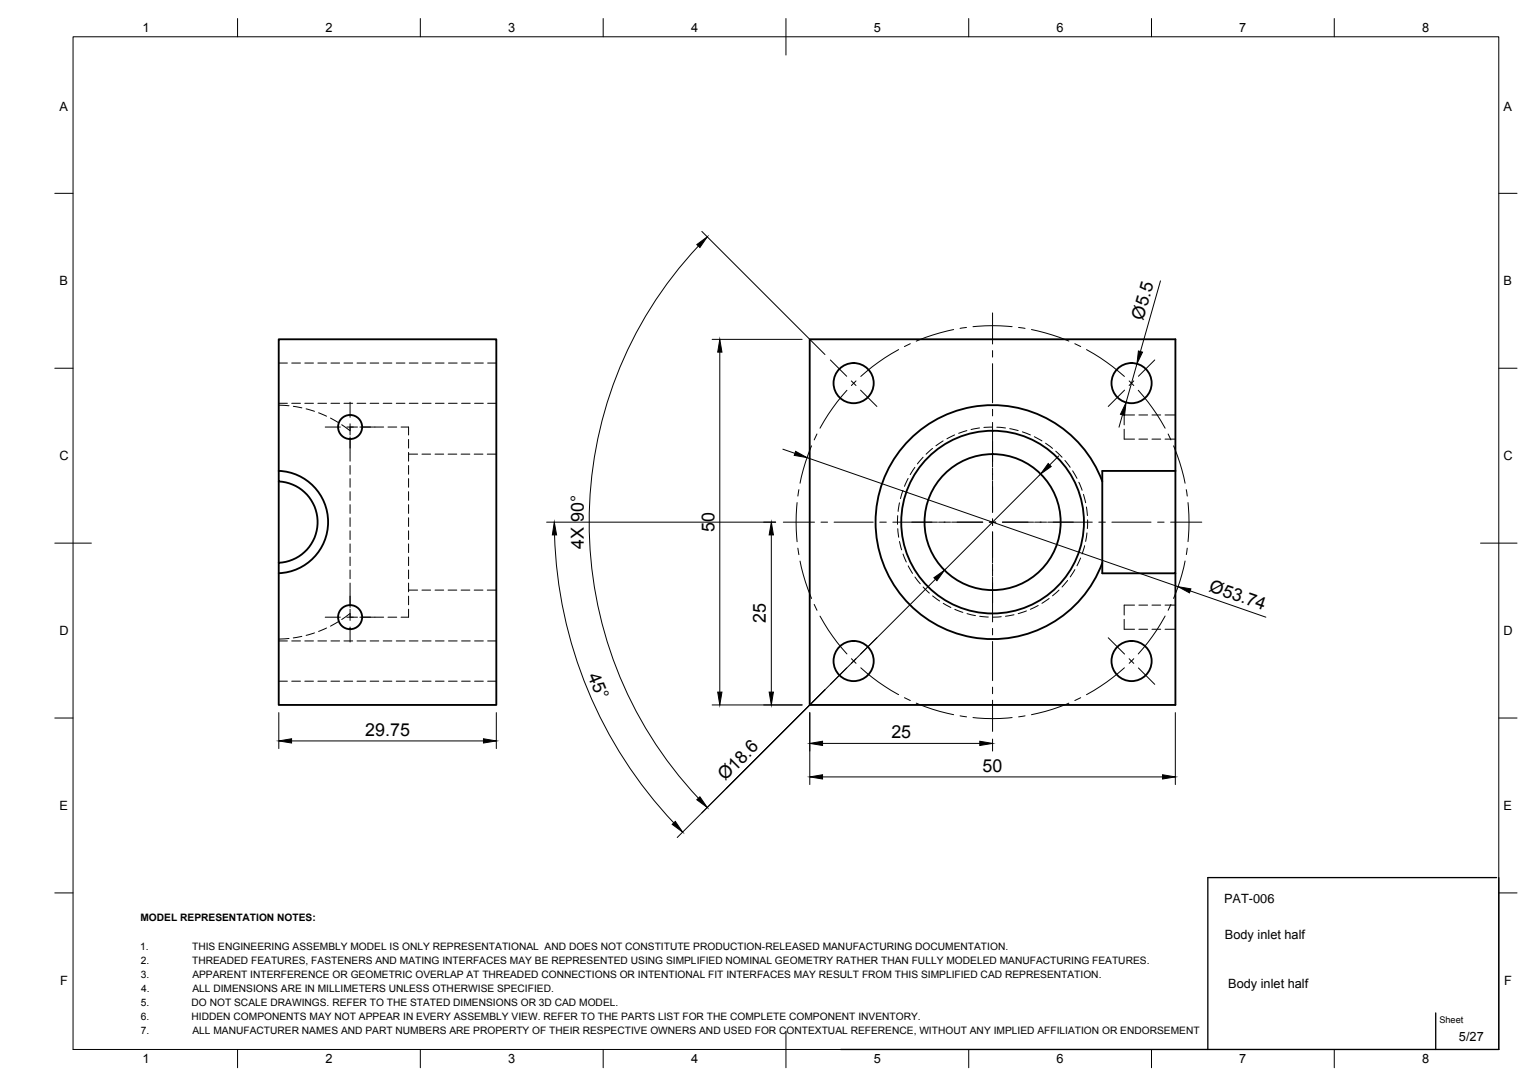
ISO-10303-21;
HEADER;
/* Generated by software containing ST-Developer
 * from STEP Tools, Inc. (www.steptools.com) 
 */

FILE_DESCRIPTION(
/* description */ ('Ball-type isolation valve (generic)'),
/* implementation_level */ '2;1');

FILE_NAME(
/* name */ 'Body inlet half.step',
/* time_stamp */ '2026-10-27T10:53:05-07:00',
/* author */ (''),
/* organization */ (''),
/* preprocessor_version */ 'ST-DEVELOPER v20.2',
/* originating_system */ 'Autodesk Translation Framework v15.17.0.0',
/* authorisation */ '');

FILE_SCHEMA (('AUTOMOTIVE_DESIGN { 1 0 10303 214 3 1 1 }'));
ENDSEC;

DATA;
#10=MECHANICAL_DESIGN_GEOMETRIC_PRESENTATION_REPRESENTATION('',(#277),#7425);
#225=SHAPE_REPRESENTATION_RELATIONSHIP('SRR','None',#7535,#251);
#251=ADVANCED_BREP_SHAPE_REPRESENTATION('',(#303),#7398);
#277=STYLED_ITEM('',(#7723),#303);
#303=MANIFOLD_SOLID_BREP('Body1',#4082);
#326=SPHERICAL_SURFACE('',#4436,1.6);
#331=FACE_BOUND('',#839,.T.);
#332=FACE_BOUND('',#840,.T.);
#333=FACE_BOUND('',#844,.T.);
#334=FACE_BOUND('',#846,.T.);
#335=FACE_BOUND('',#848,.T.);
#336=FACE_BOUND('',#850,.T.);
#337=FACE_BOUND('',#851,.T.);
#338=FACE_BOUND('',#852,.T.);
#339=FACE_BOUND('',#853,.T.);
#340=FACE_BOUND('',#856,.T.);
#341=FACE_BOUND('',#857,.T.);
#342=FACE_BOUND('',#858,.T.);
#343=FACE_BOUND('',#859,.T.);
#344=FACE_BOUND('',#860,.T.);
#419=PLANE('',#4404);
#420=PLANE('',#4408);
#421=PLANE('',#4424);
#422=PLANE('',#4426);
#423=PLANE('',#4433);
#424=PLANE('',#4435);
#425=PLANE('',#4438);
#426=PLANE('',#4439);
#427=PLANE('',#4440);
#428=PLANE('',#4441);
#429=PLANE('',#4442);
#579=FACE_OUTER_BOUND('',#828,.T.);
#580=FACE_OUTER_BOUND('',#829,.T.);
#581=FACE_OUTER_BOUND('',#830,.T.);
#582=FACE_OUTER_BOUND('',#831,.T.);
#583=FACE_OUTER_BOUND('',#832,.T.);
#584=FACE_OUTER_BOUND('',#833,.T.);
#585=FACE_OUTER_BOUND('',#834,.T.);
#586=FACE_OUTER_BOUND('',#835,.T.);
#587=FACE_OUTER_BOUND('',#836,.T.);
#588=FACE_OUTER_BOUND('',#837,.T.);
#589=FACE_OUTER_BOUND('',#838,.T.);
#590=FACE_OUTER_BOUND('',#841,.T.);
#591=FACE_OUTER_BOUND('',#842,.T.);
#592=FACE_OUTER_BOUND('',#843,.T.);
#593=FACE_OUTER_BOUND('',#845,.T.);
#594=FACE_OUTER_BOUND('',#847,.T.);
#595=FACE_OUTER_BOUND('',#849,.T.);
#596=FACE_OUTER_BOUND('',#854,.T.);
#597=FACE_OUTER_BOUND('',#855,.T.);
#598=FACE_OUTER_BOUND('',#861,.T.);
#599=FACE_OUTER_BOUND('',#862,.T.);
#828=EDGE_LOOP('',(#2775,#2776,#2777,#2778));
#829=EDGE_LOOP('',(#2779));
#830=EDGE_LOOP('',(#2780,#2781,#2782,#2783));
#831=EDGE_LOOP('',(#2784));
#832=EDGE_LOOP('',(#2785,#2786,#2787,#2788));
#833=EDGE_LOOP('',(#2789,#2790,#2791,#2792));
#834=EDGE_LOOP('',(#2793,#2794,#2795,#2796));
#835=EDGE_LOOP('',(#2797,#2798,#2799,#2800));
#836=EDGE_LOOP('',(#2801,#2802,#2803,#2804));
#837=EDGE_LOOP('',(#2805,#2806,#2807,#2808));
#838=EDGE_LOOP('',(#2809,#2810,#2811,#2812,#2813,#2814));
#839=EDGE_LOOP('',(#2815));
#840=EDGE_LOOP('',(#2816));
#841=EDGE_LOOP('',(#2817,#2818,#2819,#2820));
#842=EDGE_LOOP('',(#2821,#2822,#2823,#2824));
#843=EDGE_LOOP('',(#2825));
#844=EDGE_LOOP('',(#2826));
#845=EDGE_LOOP('',(#2827));
#846=EDGE_LOOP('',(#2828));
#847=EDGE_LOOP('',(#2829,#2830));
#848=EDGE_LOOP('',(#2831));
#849=EDGE_LOOP('',(#2832,#2833,#2834,#2835,#2836,#2837,#2838,#2839,#2840,
#2841));
#850=EDGE_LOOP('',(#2842));
#851=EDGE_LOOP('',(#2843));
#852=EDGE_LOOP('',(#2844));
#853=EDGE_LOOP('',(#2845));
#854=EDGE_LOOP('',(#2846,#2847,#2848,#2849));
#855=EDGE_LOOP('',(#2850,#2851,#2852,#2853));
#856=EDGE_LOOP('',(#2854));
#857=EDGE_LOOP('',(#2855));
#858=EDGE_LOOP('',(#2856));
#859=EDGE_LOOP('',(#2857));
#860=EDGE_LOOP('',(#2858));
#861=EDGE_LOOP('',(#2859,#2860,#2861,#2862));
#862=EDGE_LOOP('',(#2863,#2864,#2865,#2866));
#1165=LINE('',#6207,#1473);
#1166=LINE('',#6214,#1474);
#1167=LINE('',#6221,#1475);
#1168=LINE('',#6227,#1476);
#1169=LINE('',#6233,#1477);
#1170=LINE('',#6239,#1478);
#1171=LINE('',#6244,#1479);
#1172=LINE('',#6248,#1480);
#1173=LINE('',#6252,#1481);
#1174=LINE('',#6255,#1482);
#1175=LINE('',#6258,#1483);
#1176=LINE('',#6260,#1484);
#1177=LINE('',#6262,#1485);
#1178=LINE('',#6264,#1486);
#1179=LINE('',#6265,#1487);
#1180=LINE('',#6270,#1488);
#1181=LINE('',#6276,#1489);
#1182=LINE('',#6286,#1490);
#1183=LINE('',#6288,#1491);
#1184=LINE('',#6289,#1492);
#1185=LINE('',#6292,#1493);
#1186=LINE('',#6293,#1494);
#1187=LINE('',#6296,#1495);
#1188=LINE('',#6297,#1496);
#1189=LINE('',#6299,#1497);
#1473=VECTOR('',#4906,0.165);
#1474=VECTOR('',#4915,0.165);
#1475=VECTOR('',#4924,0.275);
#1476=VECTOR('',#4931,0.275);
#1477=VECTOR('',#4938,0.275);
#1478=VECTOR('',#4945,0.275);
#1479=VECTOR('',#4950,1.);
#1480=VECTOR('',#4953,1.);
#1481=VECTOR('',#4958,1.);
#1482=VECTOR('',#4961,1.);
#1483=VECTOR('',#4964,1.);
#1484=VECTOR('',#4965,1.);
#1485=VECTOR('',#4966,1.);
#1486=VECTOR('',#4967,1.);
#1487=VECTOR('',#4968,1.);
#1488=VECTOR('',#4973,0.93);
#1489=VECTOR('',#4980,1.3);
#1490=VECTOR('',#4995,1.);
#1491=VECTOR('',#4996,1.);
#1492=VECTOR('',#4997,1.);
#1493=VECTOR('',#5000,1.);
#1494=VECTOR('',#5001,1.);
#1495=VECTOR('',#5004,1.);
#1496=VECTOR('',#5005,1.);
#1497=VECTOR('',#5008,1.);
#1781=CIRCLE('',#4402,0.165);
#1782=CIRCLE('',#4403,0.165);
#1783=CIRCLE('',#4406,0.165);
#1784=CIRCLE('',#4407,0.165);
#1785=CIRCLE('',#4410,0.275);
#1786=CIRCLE('',#4411,0.275);
#1787=CIRCLE('',#4413,0.275);
#1788=CIRCLE('',#4414,0.275);
#1789=CIRCLE('',#4416,0.275);
#1790=CIRCLE('',#4417,0.275);
#1791=CIRCLE('',#4419,0.275);
#1792=CIRCLE('',#4420,0.275);
#1793=CIRCLE('',#4422,0.7);
#1794=CIRCLE('',#4423,0.7);
#1795=CIRCLE('',#4425,0.556776436283003);
#1796=CIRCLE('',#4428,0.93);
#1797=CIRCLE('',#4429,0.93);
#1798=CIRCLE('',#4431,1.3);
#1799=CIRCLE('',#4432,1.3);
#1800=CIRCLE('',#4434,1.24899959967968);
#1801=CIRCLE('',#4437,1.59980467557762);
#1956=VERTEX_POINT('',#6204);
#1957=VERTEX_POINT('',#6206);
#1958=VERTEX_POINT('',#6211);
#1959=VERTEX_POINT('',#6213);
#1960=VERTEX_POINT('',#6218);
#1961=VERTEX_POINT('',#6220);
#1962=VERTEX_POINT('',#6224);
#1963=VERTEX_POINT('',#6226);
#1964=VERTEX_POINT('',#6230);
#1965=VERTEX_POINT('',#6232);
#1966=VERTEX_POINT('',#6236);
#1967=VERTEX_POINT('',#6238);
#1968=VERTEX_POINT('',#6242);
#1969=VERTEX_POINT('',#6243);
#1970=VERTEX_POINT('',#6245);
#1971=VERTEX_POINT('',#6247);
#1972=VERTEX_POINT('',#6251);
#1973=VERTEX_POINT('',#6253);
#1974=VERTEX_POINT('',#6257);
#1975=VERTEX_POINT('',#6259);
#1976=VERTEX_POINT('',#6261);
#1977=VERTEX_POINT('',#6263);
#1978=VERTEX_POINT('',#6267);
#1979=VERTEX_POINT('',#6269);
#1980=VERTEX_POINT('',#6273);
#1981=VERTEX_POINT('',#6275);
#1982=VERTEX_POINT('',#6279);
#1983=VERTEX_POINT('',#6285);
#1984=VERTEX_POINT('',#6287);
#1985=VERTEX_POINT('',#6291);
#1986=VERTEX_POINT('',#6295);
#2280=EDGE_CURVE('',#1956,#1956,#1781,.T.);
#2281=EDGE_CURVE('',#1956,#1957,#1165,.T.);
#2282=EDGE_CURVE('',#1957,#1957,#1782,.T.);
#2283=EDGE_CURVE('',#1958,#1958,#1783,.T.);
#2284=EDGE_CURVE('',#1958,#1959,#1166,.T.);
#2285=EDGE_CURVE('',#1959,#1959,#1784,.T.);
#2286=EDGE_CURVE('',#1960,#1960,#1785,.T.);
#2287=EDGE_CURVE('',#1960,#1961,#1167,.T.);
#2288=EDGE_CURVE('',#1961,#1961,#1786,.T.);
#2289=EDGE_CURVE('',#1962,#1962,#1787,.T.);
#2290=EDGE_CURVE('',#1962,#1963,#1168,.T.);
#2291=EDGE_CURVE('',#1963,#1963,#1788,.T.);
#2292=EDGE_CURVE('',#1964,#1964,#1789,.T.);
#2293=EDGE_CURVE('',#1964,#1965,#1169,.T.);
#2294=EDGE_CURVE('',#1965,#1965,#1790,.T.);
#2295=EDGE_CURVE('',#1966,#1966,#1791,.T.);
#2296=EDGE_CURVE('',#1966,#1967,#1170,.T.);
#2297=EDGE_CURVE('',#1967,#1967,#1792,.T.);
#2298=EDGE_CURVE('',#1968,#1969,#1171,.T.);
#2299=EDGE_CURVE('',#1970,#1968,#1793,.T.);
#2300=EDGE_CURVE('',#1971,#1970,#1172,.T.);
#2301=EDGE_CURVE('',#1969,#1971,#1794,.T.);
#2302=EDGE_CURVE('',#1972,#1968,#1173,.T.);
#2303=EDGE_CURVE('',#1973,#1972,#1795,.T.);
#2304=EDGE_CURVE('',#1970,#1973,#1174,.T.);
#2305=EDGE_CURVE('',#1971,#1974,#1175,.T.);
#2306=EDGE_CURVE('',#1974,#1975,#1176,.T.);
#2307=EDGE_CURVE('',#1975,#1976,#1177,.T.);
#2308=EDGE_CURVE('',#1976,#1977,#1178,.T.);
#2309=EDGE_CURVE('',#1977,#1969,#1179,.T.);
#2310=EDGE_CURVE('',#1978,#1978,#1796,.T.);
#2311=EDGE_CURVE('',#1978,#1979,#1180,.T.);
#2312=EDGE_CURVE('',#1979,#1979,#1797,.T.);
#2313=EDGE_CURVE('',#1980,#1980,#1798,.T.);
#2314=EDGE_CURVE('',#1980,#1981,#1181,.T.);
#2315=EDGE_CURVE('',#1981,#1981,#1799,.T.);
#2316=EDGE_CURVE('',#1982,#1982,#1800,.T.);
#2317=EDGE_CURVE('',#1973,#1972,#1801,.T.);
#2318=EDGE_CURVE('',#1983,#1977,#1182,.T.);
#2319=EDGE_CURVE('',#1983,#1984,#1183,.T.);
#2320=EDGE_CURVE('',#1984,#1974,#1184,.T.);
#2321=EDGE_CURVE('',#1985,#1983,#1185,.T.);
#2322=EDGE_CURVE('',#1985,#1976,#1186,.T.);
#2323=EDGE_CURVE('',#1986,#1985,#1187,.T.);
#2324=EDGE_CURVE('',#1986,#1975,#1188,.T.);
#2325=EDGE_CURVE('',#1984,#1986,#1189,.T.);
#2775=ORIENTED_EDGE('',*,*,#2280,.F.);
#2776=ORIENTED_EDGE('',*,*,#2281,.T.);
#2777=ORIENTED_EDGE('',*,*,#2282,.F.);
#2778=ORIENTED_EDGE('',*,*,#2281,.F.);
#2779=ORIENTED_EDGE('',*,*,#2280,.T.);
#2780=ORIENTED_EDGE('',*,*,#2283,.F.);
#2781=ORIENTED_EDGE('',*,*,#2284,.T.);
#2782=ORIENTED_EDGE('',*,*,#2285,.F.);
#2783=ORIENTED_EDGE('',*,*,#2284,.F.);
#2784=ORIENTED_EDGE('',*,*,#2283,.T.);
#2785=ORIENTED_EDGE('',*,*,#2286,.F.);
#2786=ORIENTED_EDGE('',*,*,#2287,.T.);
#2787=ORIENTED_EDGE('',*,*,#2288,.F.);
#2788=ORIENTED_EDGE('',*,*,#2287,.F.);
#2789=ORIENTED_EDGE('',*,*,#2289,.F.);
#2790=ORIENTED_EDGE('',*,*,#2290,.T.);
#2791=ORIENTED_EDGE('',*,*,#2291,.F.);
#2792=ORIENTED_EDGE('',*,*,#2290,.F.);
#2793=ORIENTED_EDGE('',*,*,#2292,.F.);
#2794=ORIENTED_EDGE('',*,*,#2293,.T.);
#2795=ORIENTED_EDGE('',*,*,#2294,.F.);
#2796=ORIENTED_EDGE('',*,*,#2293,.F.);
#2797=ORIENTED_EDGE('',*,*,#2295,.F.);
#2798=ORIENTED_EDGE('',*,*,#2296,.T.);
#2799=ORIENTED_EDGE('',*,*,#2297,.F.);
#2800=ORIENTED_EDGE('',*,*,#2296,.F.);
#2801=ORIENTED_EDGE('',*,*,#2298,.F.);
#2802=ORIENTED_EDGE('',*,*,#2299,.F.);
#2803=ORIENTED_EDGE('',*,*,#2300,.F.);
#2804=ORIENTED_EDGE('',*,*,#2301,.F.);
#2805=ORIENTED_EDGE('',*,*,#2302,.F.);
#2806=ORIENTED_EDGE('',*,*,#2303,.F.);
#2807=ORIENTED_EDGE('',*,*,#2304,.F.);
#2808=ORIENTED_EDGE('',*,*,#2299,.T.);
#2809=ORIENTED_EDGE('',*,*,#2301,.T.);
#2810=ORIENTED_EDGE('',*,*,#2305,.T.);
#2811=ORIENTED_EDGE('',*,*,#2306,.T.);
#2812=ORIENTED_EDGE('',*,*,#2307,.T.);
#2813=ORIENTED_EDGE('',*,*,#2308,.T.);
#2814=ORIENTED_EDGE('',*,*,#2309,.T.);
#2815=ORIENTED_EDGE('',*,*,#2282,.T.);
#2816=ORIENTED_EDGE('',*,*,#2285,.T.);
#2817=ORIENTED_EDGE('',*,*,#2310,.F.);
#2818=ORIENTED_EDGE('',*,*,#2311,.T.);
#2819=ORIENTED_EDGE('',*,*,#2312,.F.);
#2820=ORIENTED_EDGE('',*,*,#2311,.F.);
#2821=ORIENTED_EDGE('',*,*,#2313,.F.);
#2822=ORIENTED_EDGE('',*,*,#2314,.T.);
#2823=ORIENTED_EDGE('',*,*,#2315,.T.);
#2824=ORIENTED_EDGE('',*,*,#2314,.F.);
#2825=ORIENTED_EDGE('',*,*,#2315,.F.);
#2826=ORIENTED_EDGE('',*,*,#2316,.F.);
#2827=ORIENTED_EDGE('',*,*,#2313,.T.);
#2828=ORIENTED_EDGE('',*,*,#2312,.T.);
#2829=ORIENTED_EDGE('',*,*,#2303,.T.);
#2830=ORIENTED_EDGE('',*,*,#2317,.F.);
#2831=ORIENTED_EDGE('',*,*,#2316,.T.);
#2832=ORIENTED_EDGE('',*,*,#2298,.T.);
#2833=ORIENTED_EDGE('',*,*,#2309,.F.);
#2834=ORIENTED_EDGE('',*,*,#2318,.F.);
#2835=ORIENTED_EDGE('',*,*,#2319,.T.);
#2836=ORIENTED_EDGE('',*,*,#2320,.T.);
#2837=ORIENTED_EDGE('',*,*,#2305,.F.);
#2838=ORIENTED_EDGE('',*,*,#2300,.T.);
#2839=ORIENTED_EDGE('',*,*,#2304,.T.);
#2840=ORIENTED_EDGE('',*,*,#2317,.T.);
#2841=ORIENTED_EDGE('',*,*,#2302,.T.);
#2842=ORIENTED_EDGE('',*,*,#2288,.T.);
#2843=ORIENTED_EDGE('',*,*,#2291,.T.);
#2844=ORIENTED_EDGE('',*,*,#2294,.T.);
#2845=ORIENTED_EDGE('',*,*,#2297,.T.);
#2846=ORIENTED_EDGE('',*,*,#2321,.T.);
#2847=ORIENTED_EDGE('',*,*,#2318,.T.);
#2848=ORIENTED_EDGE('',*,*,#2308,.F.);
#2849=ORIENTED_EDGE('',*,*,#2322,.F.);
#2850=ORIENTED_EDGE('',*,*,#2323,.T.);
#2851=ORIENTED_EDGE('',*,*,#2322,.T.);
#2852=ORIENTED_EDGE('',*,*,#2307,.F.);
#2853=ORIENTED_EDGE('',*,*,#2324,.F.);
#2854=ORIENTED_EDGE('',*,*,#2310,.T.);
#2855=ORIENTED_EDGE('',*,*,#2295,.T.);
#2856=ORIENTED_EDGE('',*,*,#2292,.T.);
#2857=ORIENTED_EDGE('',*,*,#2289,.T.);
#2858=ORIENTED_EDGE('',*,*,#2286,.T.);
#2859=ORIENTED_EDGE('',*,*,#2325,.T.);
#2860=ORIENTED_EDGE('',*,*,#2324,.T.);
#2861=ORIENTED_EDGE('',*,*,#2306,.F.);
#2862=ORIENTED_EDGE('',*,*,#2320,.F.);
#2863=ORIENTED_EDGE('',*,*,#2325,.F.);
#2864=ORIENTED_EDGE('',*,*,#2319,.F.);
#2865=ORIENTED_EDGE('',*,*,#2321,.F.);
#2866=ORIENTED_EDGE('',*,*,#2323,.F.);
#3765=CYLINDRICAL_SURFACE('',#4401,0.165);
#3766=CYLINDRICAL_SURFACE('',#4405,0.165);
#3767=CYLINDRICAL_SURFACE('',#4409,0.275);
#3768=CYLINDRICAL_SURFACE('',#4412,0.275);
#3769=CYLINDRICAL_SURFACE('',#4415,0.275);
#3770=CYLINDRICAL_SURFACE('',#4418,0.275);
#3771=CYLINDRICAL_SURFACE('',#4421,0.7);
#3772=CYLINDRICAL_SURFACE('',#4427,0.93);
#3773=CYLINDRICAL_SURFACE('',#4430,1.3);
#3833=ADVANCED_FACE('',(#579),#3765,.F.);
#3834=ADVANCED_FACE('',(#580),#419,.T.);
#3835=ADVANCED_FACE('',(#581),#3766,.F.);
#3836=ADVANCED_FACE('',(#582),#420,.T.);
#3837=ADVANCED_FACE('',(#583),#3767,.F.);
#3838=ADVANCED_FACE('',(#584),#3768,.F.);
#3839=ADVANCED_FACE('',(#585),#3769,.F.);
#3840=ADVANCED_FACE('',(#586),#3770,.F.);
#3841=ADVANCED_FACE('',(#587),#3771,.F.);
#3842=ADVANCED_FACE('',(#588),#421,.T.);
#3843=ADVANCED_FACE('',(#589,#331,#332),#422,.T.);
#3844=ADVANCED_FACE('',(#590),#3772,.F.);
#3845=ADVANCED_FACE('',(#591),#3773,.F.);
#3846=ADVANCED_FACE('',(#592,#333),#423,.F.);
#3847=ADVANCED_FACE('',(#593,#334),#424,.T.);
#3848=ADVANCED_FACE('',(#594,#335),#326,.F.);
#3849=ADVANCED_FACE('',(#595,#336,#337,#338,#339),#425,.T.);
#3850=ADVANCED_FACE('',(#596),#426,.T.);
#3851=ADVANCED_FACE('',(#597,#340,#341,#342,#343,#344),#427,.T.);
#3852=ADVANCED_FACE('',(#598),#428,.T.);
#3853=ADVANCED_FACE('',(#599),#429,.F.);
#4082=CLOSED_SHELL('',(#3833,#3834,#3835,#3836,#3837,#3838,#3839,#3840,
#3841,#3842,#3843,#3844,#3845,#3846,#3847,#3848,#3849,#3850,#3851,#3852,
#3853));
#4400=AXIS2_PLACEMENT_3D('',#6202,#4900,#4901);
#4401=AXIS2_PLACEMENT_3D('',#6203,#4902,#4903);
#4402=AXIS2_PLACEMENT_3D('',#6205,#4904,#4905);
#4403=AXIS2_PLACEMENT_3D('',#6208,#4907,#4908);
#4404=AXIS2_PLACEMENT_3D('',#6209,#4909,#4910);
#4405=AXIS2_PLACEMENT_3D('',#6210,#4911,#4912);
#4406=AXIS2_PLACEMENT_3D('',#6212,#4913,#4914);
#4407=AXIS2_PLACEMENT_3D('',#6215,#4916,#4917);
#4408=AXIS2_PLACEMENT_3D('',#6216,#4918,#4919);
#4409=AXIS2_PLACEMENT_3D('',#6217,#4920,#4921);
#4410=AXIS2_PLACEMENT_3D('',#6219,#4922,#4923);
#4411=AXIS2_PLACEMENT_3D('',#6222,#4925,#4926);
#4412=AXIS2_PLACEMENT_3D('',#6223,#4927,#4928);
#4413=AXIS2_PLACEMENT_3D('',#6225,#4929,#4930);
#4414=AXIS2_PLACEMENT_3D('',#6228,#4932,#4933);
#4415=AXIS2_PLACEMENT_3D('',#6229,#4934,#4935);
#4416=AXIS2_PLACEMENT_3D('',#6231,#4936,#4937);
#4417=AXIS2_PLACEMENT_3D('',#6234,#4939,#4940);
#4418=AXIS2_PLACEMENT_3D('',#6235,#4941,#4942);
#4419=AXIS2_PLACEMENT_3D('',#6237,#4943,#4944);
#4420=AXIS2_PLACEMENT_3D('',#6240,#4946,#4947);
#4421=AXIS2_PLACEMENT_3D('',#6241,#4948,#4949);
#4422=AXIS2_PLACEMENT_3D('',#6246,#4951,#4952);
#4423=AXIS2_PLACEMENT_3D('',#6249,#4954,#4955);
#4424=AXIS2_PLACEMENT_3D('',#6250,#4956,#4957);
#4425=AXIS2_PLACEMENT_3D('',#6254,#4959,#4960);
#4426=AXIS2_PLACEMENT_3D('',#6256,#4962,#4963);
#4427=AXIS2_PLACEMENT_3D('',#6266,#4969,#4970);
#4428=AXIS2_PLACEMENT_3D('',#6268,#4971,#4972);
#4429=AXIS2_PLACEMENT_3D('',#6271,#4974,#4975);
#4430=AXIS2_PLACEMENT_3D('',#6272,#4976,#4977);
#4431=AXIS2_PLACEMENT_3D('',#6274,#4978,#4979);
#4432=AXIS2_PLACEMENT_3D('',#6277,#4981,#4982);
#4433=AXIS2_PLACEMENT_3D('',#6278,#4983,#4984);
#4434=AXIS2_PLACEMENT_3D('',#6280,#4985,#4986);
#4435=AXIS2_PLACEMENT_3D('',#6281,#4987,#4988);
#4436=AXIS2_PLACEMENT_3D('',#6282,#4989,#4990);
#4437=AXIS2_PLACEMENT_3D('',#6283,#4991,#4992);
#4438=AXIS2_PLACEMENT_3D('',#6284,#4993,#4994);
#4439=AXIS2_PLACEMENT_3D('',#6290,#4998,#4999);
#4440=AXIS2_PLACEMENT_3D('',#6294,#5002,#5003);
#4441=AXIS2_PLACEMENT_3D('',#6298,#5006,#5007);
#4442=AXIS2_PLACEMENT_3D('',#6300,#5009,#5010);
#4900=DIRECTION('axis',(0.,0.,1.));
#4901=DIRECTION('refdir',(1.,0.,0.));
#4902=DIRECTION('center_axis',(0.,0.,1.));
#4903=DIRECTION('ref_axis',(1.,0.,0.));
#4904=DIRECTION('center_axis',(0.,0.,1.));
#4905=DIRECTION('ref_axis',(1.,0.,0.));
#4906=DIRECTION('',(0.,0.,1.));
#4907=DIRECTION('center_axis',(0.,0.,-1.));
#4908=DIRECTION('ref_axis',(1.,0.,0.));
#4909=DIRECTION('center_axis',(0.,0.,1.));
#4910=DIRECTION('ref_axis',(1.,0.,0.));
#4911=DIRECTION('center_axis',(0.,0.,1.));
#4912=DIRECTION('ref_axis',(1.,0.,0.));
#4913=DIRECTION('center_axis',(0.,0.,1.));
#4914=DIRECTION('ref_axis',(1.,0.,0.));
#4915=DIRECTION('',(0.,0.,1.));
#4916=DIRECTION('center_axis',(0.,0.,-1.));
#4917=DIRECTION('ref_axis',(1.,0.,0.));
#4918=DIRECTION('center_axis',(0.,0.,1.));
#4919=DIRECTION('ref_axis',(1.,0.,0.));
#4920=DIRECTION('center_axis',(0.,1.,0.));
#4921=DIRECTION('ref_axis',(1.,0.,0.));
#4922=DIRECTION('center_axis',(0.,1.,0.));
#4923=DIRECTION('ref_axis',(1.,0.,0.));
#4924=DIRECTION('',(0.,1.,0.));
#4925=DIRECTION('center_axis',(0.,-1.,0.));
#4926=DIRECTION('ref_axis',(1.,0.,0.));
#4927=DIRECTION('center_axis',(0.,1.,0.));
#4928=DIRECTION('ref_axis',(1.,0.,0.));
#4929=DIRECTION('center_axis',(0.,1.,0.));
#4930=DIRECTION('ref_axis',(1.,0.,0.));
#4931=DIRECTION('',(0.,1.,0.));
#4932=DIRECTION('center_axis',(0.,-1.,0.));
#4933=DIRECTION('ref_axis',(1.,0.,0.));
#4934=DIRECTION('center_axis',(0.,1.,0.));
#4935=DIRECTION('ref_axis',(1.,0.,0.));
#4936=DIRECTION('center_axis',(0.,1.,0.));
#4937=DIRECTION('ref_axis',(1.,0.,0.));
#4938=DIRECTION('',(0.,1.,0.));
#4939=DIRECTION('center_axis',(0.,-1.,0.));
#4940=DIRECTION('ref_axis',(1.,0.,0.));
#4941=DIRECTION('center_axis',(0.,1.,0.));
#4942=DIRECTION('ref_axis',(1.,0.,0.));
#4943=DIRECTION('center_axis',(0.,1.,0.));
#4944=DIRECTION('ref_axis',(1.,0.,0.));
#4945=DIRECTION('',(0.,1.,0.));
#4946=DIRECTION('center_axis',(0.,-1.,0.));
#4947=DIRECTION('ref_axis',(1.,0.,0.));
#4948=DIRECTION('center_axis',(0.,0.,1.));
#4949=DIRECTION('ref_axis',(1.,0.,0.));
#4950=DIRECTION('',(0.,0.,1.));
#4951=DIRECTION('center_axis',(0.,0.,1.));
#4952=DIRECTION('ref_axis',(1.,0.,0.));
#4953=DIRECTION('',(0.,0.,-1.));
#4954=DIRECTION('center_axis',(0.,0.,-1.));
#4955=DIRECTION('ref_axis',(1.,0.,0.));
#4956=DIRECTION('center_axis',(0.,0.,1.));
#4957=DIRECTION('ref_axis',(1.,0.,0.));
#4958=DIRECTION('',(1.,0.,0.));
#4959=DIRECTION('center_axis',(0.,0.,1.));
#4960=DIRECTION('ref_axis',(0.,-1.,0.));
#4961=DIRECTION('',(1.,0.,0.));
#4962=DIRECTION('center_axis',(0.,0.,1.));
#4963=DIRECTION('ref_axis',(1.,0.,0.));
#4964=DIRECTION('',(-1.,0.,0.));
#4965=DIRECTION('',(0.,-1.,0.));
#4966=DIRECTION('',(1.,0.,0.));
#4967=DIRECTION('',(0.,1.,0.));
#4968=DIRECTION('',(-1.,0.,0.));
#4969=DIRECTION('center_axis',(0.,1.,0.));
#4970=DIRECTION('ref_axis',(1.,0.,0.));
#4971=DIRECTION('center_axis',(0.,1.,0.));
#4972=DIRECTION('ref_axis',(1.,0.,0.));
#4973=DIRECTION('',(0.,1.,0.));
#4974=DIRECTION('center_axis',(0.,-1.,0.));
#4975=DIRECTION('ref_axis',(1.,0.,0.));
#4976=DIRECTION('center_axis',(0.,1.,0.));
#4977=DIRECTION('ref_axis',(1.,0.,0.));
#4978=DIRECTION('center_axis',(0.,1.,0.));
#4979=DIRECTION('ref_axis',(1.,0.,0.));
#4980=DIRECTION('',(0.,1.,0.));
#4981=DIRECTION('center_axis',(0.,1.,0.));
#4982=DIRECTION('ref_axis',(1.,0.,0.));
#4983=DIRECTION('center_axis',(0.,1.,0.));
#4984=DIRECTION('ref_axis',(1.,0.,0.));
#4985=DIRECTION('center_axis',(0.,-1.,0.));
#4986=DIRECTION('ref_axis',(0.,0.,-1.));
#4987=DIRECTION('center_axis',(0.,1.,0.));
#4988=DIRECTION('ref_axis',(1.,0.,0.));
#4989=DIRECTION('center_axis',(6.12323399573677E-17,0.,1.));
#4990=DIRECTION('ref_axis',(1.,0.,0.));
#4991=DIRECTION('center_axis',(0.,-1.,0.));
#4992=DIRECTION('ref_axis',(0.,0.,-1.));
#4993=DIRECTION('center_axis',(0.,1.,0.));
#4994=DIRECTION('ref_axis',(-1.,0.,0.));
#4995=DIRECTION('',(0.,0.,1.));
#4996=DIRECTION('',(-1.,0.,0.));
#4997=DIRECTION('',(0.,0.,1.));
#4998=DIRECTION('center_axis',(1.,0.,0.));
#4999=DIRECTION('ref_axis',(0.,1.,0.));
#5000=DIRECTION('',(0.,1.,0.));
#5001=DIRECTION('',(0.,0.,1.));
#5002=DIRECTION('center_axis',(0.,-1.,0.));
#5003=DIRECTION('ref_axis',(1.,0.,0.));
#5004=DIRECTION('',(1.,0.,0.));
#5005=DIRECTION('',(0.,0.,1.));
#5006=DIRECTION('center_axis',(-1.,0.,0.));
#5007=DIRECTION('ref_axis',(0.,-1.,0.));
#5008=DIRECTION('',(0.,-1.,0.));
#5009=DIRECTION('center_axis',(0.,0.,1.));
#5010=DIRECTION('ref_axis',(1.,0.,0.));
#6202=CARTESIAN_POINT('',(0.,0.,0.));
#6203=CARTESIAN_POINT('Origin',(-1.3,-1.,6.8));
#6204=CARTESIAN_POINT('',(-1.465,-1.,6.8));
#6205=CARTESIAN_POINT('Origin',(-1.3,-1.,6.8));
#6206=CARTESIAN_POINT('',(-1.465,-1.,7.5));
#6207=CARTESIAN_POINT('',(-1.465,-1.,6.8));
#6208=CARTESIAN_POINT('Origin',(-1.3,-1.,7.5));
#6209=CARTESIAN_POINT('Origin',(-1.3,-1.,6.8));
#6210=CARTESIAN_POINT('Origin',(1.3,-1.,6.8));
#6211=CARTESIAN_POINT('',(1.135,-1.,6.8));
#6212=CARTESIAN_POINT('Origin',(1.3,-1.,6.8));
#6213=CARTESIAN_POINT('',(1.135,-1.,7.5));
#6214=CARTESIAN_POINT('',(1.135,-1.,6.8));
#6215=CARTESIAN_POINT('Origin',(1.3,-1.,7.5));
#6216=CARTESIAN_POINT('Origin',(1.3,-1.,6.8));
#6217=CARTESIAN_POINT('Origin',(1.9,-3.1,3.1));
#6218=CARTESIAN_POINT('',(1.625,-3.,3.1));
#6219=CARTESIAN_POINT('Origin',(1.9,-3.,3.1));
#6220=CARTESIAN_POINT('',(1.625,-0.0249999999999999,3.1));
#6221=CARTESIAN_POINT('',(1.625,-3.1,3.1));
#6222=CARTESIAN_POINT('Origin',(1.9,-0.0249999999999999,3.1));
#6223=CARTESIAN_POINT('Origin',(-1.9,-3.1,6.9));
#6224=CARTESIAN_POINT('',(-2.175,-3.,6.9));
#6225=CARTESIAN_POINT('Origin',(-1.9,-3.,6.9));
#6226=CARTESIAN_POINT('',(-2.175,-0.0249999999999999,6.9));
#6227=CARTESIAN_POINT('',(-2.175,-3.1,6.9));
#6228=CARTESIAN_POINT('Origin',(-1.9,-0.0249999999999999,6.9));
#6229=CARTESIAN_POINT('Origin',(-1.9,-3.1,3.1));
#6230=CARTESIAN_POINT('',(-2.175,-3.,3.1));
#6231=CARTESIAN_POINT('Origin',(-1.9,-3.,3.1));
#6232=CARTESIAN_POINT('',(-2.175,-0.0249999999999999,3.1));
#6233=CARTESIAN_POINT('',(-2.175,-3.1,3.1));
#6234=CARTESIAN_POINT('Origin',(-1.9,-0.0249999999999999,3.1));
#6235=CARTESIAN_POINT('Origin',(1.9,-3.1,6.9));
#6236=CARTESIAN_POINT('',(1.625,-3.,6.9));
#6237=CARTESIAN_POINT('Origin',(1.9,-3.,6.9));
#6238=CARTESIAN_POINT('',(1.625,-0.0249999999999999,6.9));
#6239=CARTESIAN_POINT('',(1.625,-3.1,6.9));
#6240=CARTESIAN_POINT('Origin',(1.9,-0.0249999999999999,6.9));
#6241=CARTESIAN_POINT('Origin',(0.,0.,6.5));
#6242=CARTESIAN_POINT('',(0.699553428981661,-0.025,6.5));
#6243=CARTESIAN_POINT('',(0.699553428981661,-0.025,7.5));
#6244=CARTESIAN_POINT('',(0.699553428981661,-0.025,6.5));
#6245=CARTESIAN_POINT('',(-0.699553428981661,-0.025,6.5));
#6246=CARTESIAN_POINT('Origin',(0.,0.,6.5));
#6247=CARTESIAN_POINT('',(-0.699553428981661,-0.025,7.5));
#6248=CARTESIAN_POINT('',(-0.699553428981661,-0.025,6.5));
#6249=CARTESIAN_POINT('Origin',(0.,0.,7.5));
#6250=CARTESIAN_POINT('Origin',(0.,0.,6.5));
#6251=CARTESIAN_POINT('',(0.556214886532175,-0.025,6.5));
#6252=CARTESIAN_POINT('',(1.25,-0.025,6.5));
#6253=CARTESIAN_POINT('',(-0.556214886532175,-0.025,6.5));
#6254=CARTESIAN_POINT('Origin',(0.,0.,6.5));
#6255=CARTESIAN_POINT('',(1.25,-0.025,6.5));
#6256=CARTESIAN_POINT('Origin',(0.,-1.5125,7.5));
#6257=CARTESIAN_POINT('',(-2.5,-0.025,7.5));
#6258=CARTESIAN_POINT('',(2.5,-0.025,7.5));
#6259=CARTESIAN_POINT('',(-2.5,-3.,7.5));
#6260=CARTESIAN_POINT('',(-2.5,-0.025,7.5));
#6261=CARTESIAN_POINT('',(2.5,-3.,7.5));
#6262=CARTESIAN_POINT('',(-2.5,-3.,7.5));
#6263=CARTESIAN_POINT('',(2.5,-0.025,7.5));
#6264=CARTESIAN_POINT('',(2.5,-3.,7.5));
#6265=CARTESIAN_POINT('',(2.5,-0.025,7.5));
#6266=CARTESIAN_POINT('Origin',(0.,-3.1,5.));
#6267=CARTESIAN_POINT('',(-0.93,-3.,5.));
#6268=CARTESIAN_POINT('Origin',(0.,-3.,5.));
#6269=CARTESIAN_POINT('',(-0.93,-1.8,5.));
#6270=CARTESIAN_POINT('',(-0.93,-3.1,5.));
#6271=CARTESIAN_POINT('Origin',(0.,-1.8,5.));
#6272=CARTESIAN_POINT('Origin',(0.,-1.8,5.));
#6273=CARTESIAN_POINT('',(-1.3,-1.8,5.));
#6274=CARTESIAN_POINT('Origin',(0.,-1.8,5.));
#6275=CARTESIAN_POINT('',(-1.3,-1.,5.));
#6276=CARTESIAN_POINT('',(-1.3,-1.8,5.));
#6277=CARTESIAN_POINT('Origin',(0.,-1.,5.));
#6278=CARTESIAN_POINT('Origin',(0.,-1.,5.));
#6279=CARTESIAN_POINT('',(-1.52958336188405E-16,-1.,6.24899959967968));
#6280=CARTESIAN_POINT('Origin',(0.,-1.,5.));
#6281=CARTESIAN_POINT('Origin',(0.,-1.8,5.));
#6282=CARTESIAN_POINT('Origin',(0.,0.,5.));
#6283=CARTESIAN_POINT('Origin',(0.,-0.025,5.));
#6284=CARTESIAN_POINT('Origin',(2.5,-0.025,2.5));
#6285=CARTESIAN_POINT('',(2.5,-0.025,2.5));
#6286=CARTESIAN_POINT('',(2.5,-0.025,2.5));
#6287=CARTESIAN_POINT('',(-2.5,-0.025,2.5));
#6288=CARTESIAN_POINT('',(2.5,-0.025,2.5));
#6289=CARTESIAN_POINT('',(-2.5,-0.025,2.5));
#6290=CARTESIAN_POINT('Origin',(2.5,-3.,2.5));
#6291=CARTESIAN_POINT('',(2.5,-3.,2.5));
#6292=CARTESIAN_POINT('',(2.5,-3.,2.5));
#6293=CARTESIAN_POINT('',(2.5,-3.,2.5));
#6294=CARTESIAN_POINT('Origin',(-2.5,-3.,2.5));
#6295=CARTESIAN_POINT('',(-2.5,-3.,2.5));
#6296=CARTESIAN_POINT('',(-2.5,-3.,2.5));
#6297=CARTESIAN_POINT('',(-2.5,-3.,2.5));
#6298=CARTESIAN_POINT('Origin',(-2.5,-0.025,2.5));
#6299=CARTESIAN_POINT('',(-2.5,-0.025,2.5));
#6300=CARTESIAN_POINT('Origin',(0.,-1.5125,2.5));
#7368=UNCERTAINTY_MEASURE_WITH_UNIT(LENGTH_MEASURE(0.001),#7426,
'DISTANCE_ACCURACY_VALUE',
'Maximum model space distance between geometric entities at asserted c
onnectivities');
#7395=UNCERTAINTY_MEASURE_WITH_UNIT(LENGTH_MEASURE(0.001),#7426,
'DISTANCE_ACCURACY_VALUE',
'Maximum model space distance between geometric entities at asserted c
onnectivities');
#7398=(
GEOMETRIC_REPRESENTATION_CONTEXT(3)
GLOBAL_UNCERTAINTY_ASSIGNED_CONTEXT((#7368))
GLOBAL_UNIT_ASSIGNED_CONTEXT((#7426,#7428,#7429))
REPRESENTATION_CONTEXT('','3D')
);
#7425=(
GEOMETRIC_REPRESENTATION_CONTEXT(3)
GLOBAL_UNCERTAINTY_ASSIGNED_CONTEXT((#7395))
GLOBAL_UNIT_ASSIGNED_CONTEXT((#7426,#7428,#7429))
REPRESENTATION_CONTEXT('','3D')
);
#7426=(
LENGTH_UNIT()
NAMED_UNIT(*)
SI_UNIT(.CENTI.,.METRE.)
);
#7428=(
NAMED_UNIT(*)
PLANE_ANGLE_UNIT()
SI_UNIT($,.RADIAN.)
);
#7429=(
NAMED_UNIT(*)
SI_UNIT($,.STERADIAN.)
SOLID_ANGLE_UNIT()
);
#7432=SHAPE_DEFINITION_REPRESENTATION(#7461,#7535);
#7461=PRODUCT_DEFINITION_SHAPE('',$,#7565);
#7535=SHAPE_REPRESENTATION('',(#4400),#7398);
#7562=PRODUCT_DEFINITION_CONTEXT('part definition',#7651,'design');
#7565=PRODUCT_DEFINITION('Body inlet half','Body inlet half',#7594,#7562);
#7594=PRODUCT_DEFINITION_FORMATION('',$,#7655);
#7651=APPLICATION_CONTEXT(
'Core Data for Automotive Mechanical Design Process');
#7652=PRODUCT_CONTEXT('part definition',#7651,'mechanical');
#7655=PRODUCT('Body inlet half','Body inlet half','Body inlet half',(#7652));
#7717=COLOUR_RGB('Dark Blue',0.08,0.2,0.34);
#7718=FILL_AREA_STYLE_COLOUR('',#7717);
#7719=FILL_AREA_STYLE('',(#7718));
#7720=SURFACE_STYLE_FILL_AREA(#7719);
#7721=SURFACE_SIDE_STYLE('',(#7720));
#7722=SURFACE_STYLE_USAGE(.BOTH.,#7721);
#7723=PRESENTATION_STYLE_ASSIGNMENT((#7722));
ENDSEC;
END-ISO-10303-21;
